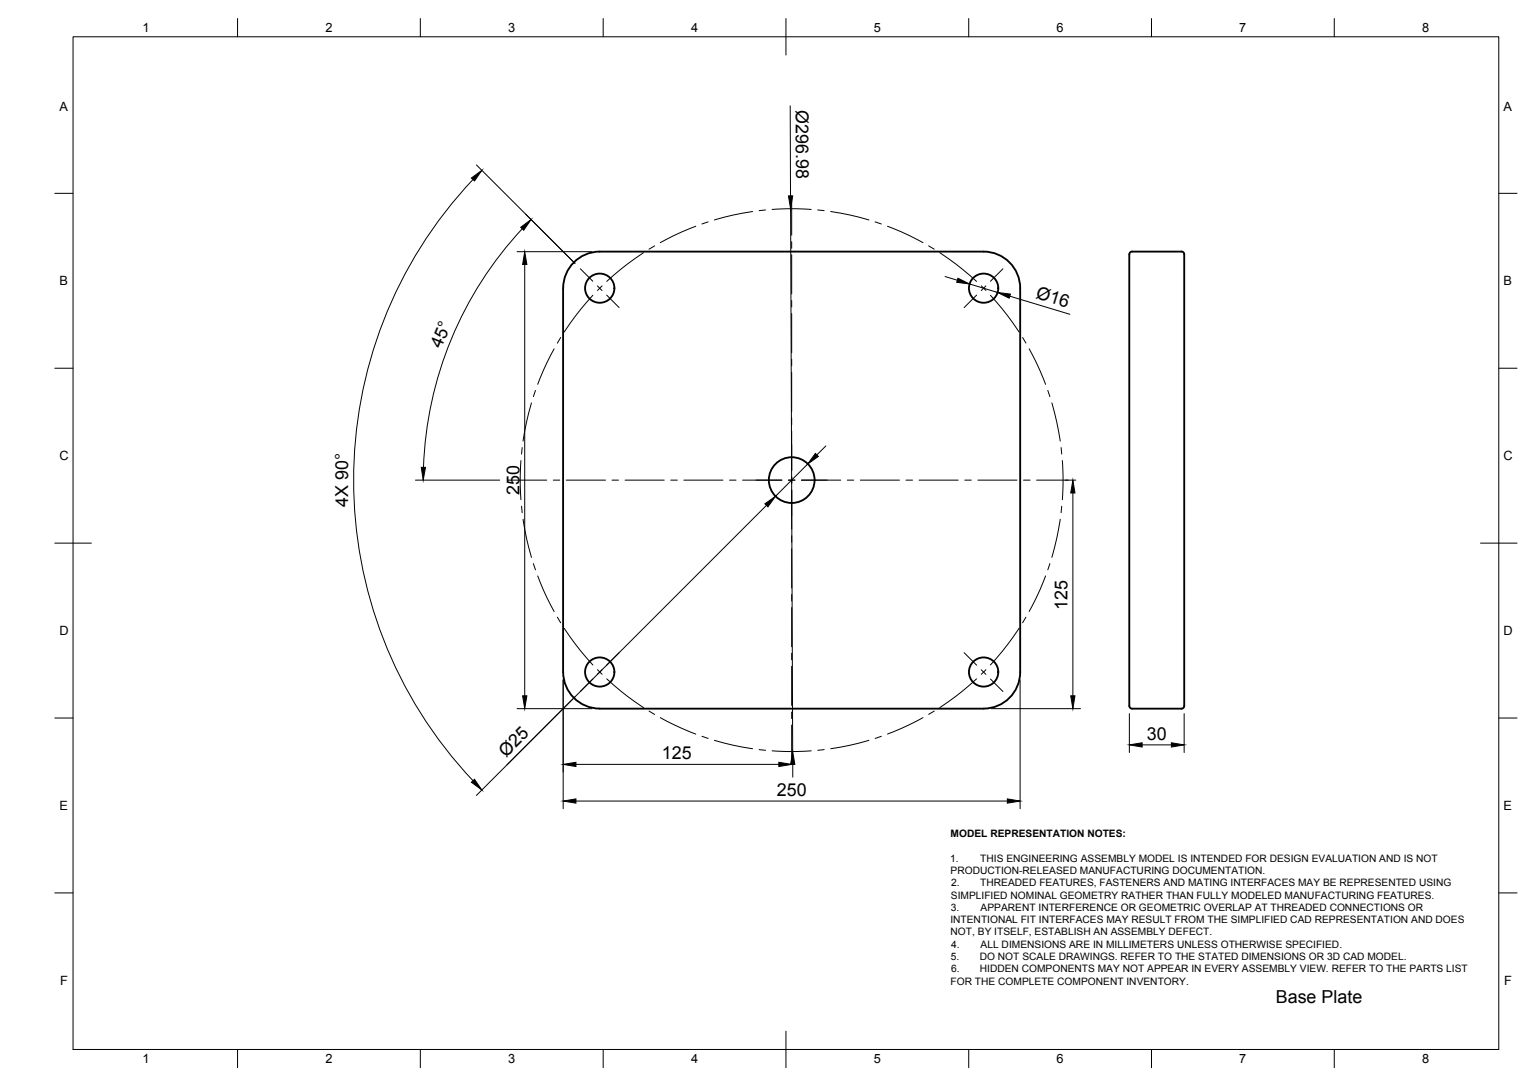
ISO-10303-21;
HEADER;
/* Generated by software containing ST-Developer
 * from STEP Tools, Inc. (www.steptools.com) 
 */

FILE_DESCRIPTION(
/* description */ ('STEP AP214'),
/* implementation_level */ '2;1');

FILE_NAME(
/* name */ 'BASE PLATE.step',
/* time_stamp */ '2026-10-06T11:20:11-07:00',
/* author */ (''),
/* organization */ (''),
/* preprocessor_version */ 'ST-DEVELOPER v20.2',
/* originating_system */ 'Autodesk Translation Framework v15.15.0.0',
/* authorisation */ '');

FILE_SCHEMA (('AUTOMOTIVE_DESIGN { 1 0 10303 214 3 1 1 }'));
ENDSEC;

DATA;
#10=MECHANICAL_DESIGN_GEOMETRIC_PRESENTATION_REPRESENTATION('',(#47),#2840);
#35=SHAPE_REPRESENTATION_RELATIONSHIP('SRR','None',#2866,#41);
#41=ADVANCED_BREP_SHAPE_REPRESENTATION('',(#53),#2834);
#47=STYLED_ITEM('',(#2905),#53);
#53=MANIFOLD_SOLID_BREP('Body1',#1547);
#59=TOROIDAL_SURFACE('',#1663,18.5,1.5);
#60=TOROIDAL_SURFACE('',#1670,18.5,1.5);
#61=TOROIDAL_SURFACE('',#1672,18.5,1.5);
#62=TOROIDAL_SURFACE('',#1678,18.5,1.5);
#63=TOROIDAL_SURFACE('',#1679,18.5,1.5);
#64=TOROIDAL_SURFACE('',#1686,18.5,1.5);
#65=TOROIDAL_SURFACE('',#1688,18.5,1.5);
#66=TOROIDAL_SURFACE('',#1694,18.5,1.5);
#70=FACE_BOUND('',#226,.T.);
#71=FACE_BOUND('',#227,.T.);
#72=FACE_BOUND('',#228,.T.);
#73=FACE_BOUND('',#229,.T.);
#74=FACE_BOUND('',#230,.T.);
#75=FACE_BOUND('',#232,.T.);
#76=FACE_BOUND('',#233,.T.);
#77=FACE_BOUND('',#234,.T.);
#78=FACE_BOUND('',#235,.T.);
#98=PLANE('',#1637);
#99=PLANE('',#1638);
#100=PLANE('',#1639);
#101=PLANE('',#1640);
#102=PLANE('',#1641);
#103=PLANE('',#1646);
#104=PLANE('',#1695);
#126=FACE_OUTER_BOUND('',#216,.T.);
#127=FACE_OUTER_BOUND('',#217,.T.);
#128=FACE_OUTER_BOUND('',#218,.T.);
#129=FACE_OUTER_BOUND('',#219,.T.);
#130=FACE_OUTER_BOUND('',#220,.T.);
#131=FACE_OUTER_BOUND('',#221,.T.);
#132=FACE_OUTER_BOUND('',#222,.T.);
#133=FACE_OUTER_BOUND('',#223,.T.);
#134=FACE_OUTER_BOUND('',#224,.T.);
#135=FACE_OUTER_BOUND('',#225,.T.);
#136=FACE_OUTER_BOUND('',#231,.T.);
#137=FACE_OUTER_BOUND('',#236,.T.);
#138=FACE_OUTER_BOUND('',#237,.T.);
#139=FACE_OUTER_BOUND('',#238,.T.);
#140=FACE_OUTER_BOUND('',#239,.T.);
#141=FACE_OUTER_BOUND('',#240,.T.);
#142=FACE_OUTER_BOUND('',#241,.T.);
#143=FACE_OUTER_BOUND('',#242,.T.);
#144=FACE_OUTER_BOUND('',#243,.T.);
#145=FACE_OUTER_BOUND('',#244,.T.);
#146=FACE_OUTER_BOUND('',#245,.T.);
#147=FACE_OUTER_BOUND('',#246,.T.);
#148=FACE_OUTER_BOUND('',#247,.T.);
#149=FACE_OUTER_BOUND('',#248,.T.);
#150=FACE_OUTER_BOUND('',#249,.T.);
#151=FACE_OUTER_BOUND('',#250,.T.);
#152=FACE_OUTER_BOUND('',#251,.T.);
#153=FACE_OUTER_BOUND('',#252,.T.);
#154=FACE_OUTER_BOUND('',#253,.T.);
#155=FACE_OUTER_BOUND('',#254,.T.);
#156=FACE_OUTER_BOUND('',#255,.T.);
#157=FACE_OUTER_BOUND('',#256,.T.);
#216=EDGE_LOOP('',(#984,#985,#986,#987));
#217=EDGE_LOOP('',(#988,#989,#990,#991));
#218=EDGE_LOOP('',(#992,#993,#994,#995));
#219=EDGE_LOOP('',(#996,#997,#998,#999));
#220=EDGE_LOOP('',(#1000,#1001,#1002,#1003));
#221=EDGE_LOOP('',(#1004,#1005,#1006,#1007));
#222=EDGE_LOOP('',(#1008,#1009,#1010,#1011));
#223=EDGE_LOOP('',(#1012,#1013,#1014,#1015));
#224=EDGE_LOOP('',(#1016,#1017,#1018,#1019));
#225=EDGE_LOOP('',(#1020,#1021,#1022,#1023,#1024,#1025,#1026,#1027));
#226=EDGE_LOOP('',(#1028));
#227=EDGE_LOOP('',(#1029));
#228=EDGE_LOOP('',(#1030));
#229=EDGE_LOOP('',(#1031));
#230=EDGE_LOOP('',(#1032));
#231=EDGE_LOOP('',(#1033,#1034,#1035,#1036,#1037,#1038,#1039,#1040));
#232=EDGE_LOOP('',(#1041));
#233=EDGE_LOOP('',(#1042));
#234=EDGE_LOOP('',(#1043));
#235=EDGE_LOOP('',(#1044));
#236=EDGE_LOOP('',(#1045,#1046,#1047,#1048));
#237=EDGE_LOOP('',(#1049,#1050,#1051,#1052));
#238=EDGE_LOOP('',(#1053,#1054,#1055,#1056));
#239=EDGE_LOOP('',(#1057,#1058,#1059,#1060));
#240=EDGE_LOOP('',(#1061,#1062,#1063,#1064));
#241=EDGE_LOOP('',(#1065,#1066,#1067,#1068));
#242=EDGE_LOOP('',(#1069,#1070,#1071,#1072));
#243=EDGE_LOOP('',(#1073,#1074,#1075,#1076));
#244=EDGE_LOOP('',(#1077,#1078,#1079,#1080));
#245=EDGE_LOOP('',(#1081,#1082,#1083,#1084));
#246=EDGE_LOOP('',(#1085,#1086,#1087,#1088));
#247=EDGE_LOOP('',(#1089,#1090,#1091,#1092));
#248=EDGE_LOOP('',(#1093,#1094,#1095,#1096));
#249=EDGE_LOOP('',(#1097,#1098,#1099,#1100));
#250=EDGE_LOOP('',(#1101,#1102,#1103,#1104));
#251=EDGE_LOOP('',(#1105,#1106,#1107,#1108));
#252=EDGE_LOOP('',(#1109,#1110,#1111,#1112));
#253=EDGE_LOOP('',(#1113,#1114,#1115,#1116));
#254=EDGE_LOOP('',(#1117,#1118,#1119,#1120));
#255=EDGE_LOOP('',(#1121,#1122,#1123,#1124));
#256=EDGE_LOOP('',(#1125));
#334=LINE('',#2382,#427);
#335=LINE('',#2388,#428);
#336=LINE('',#2394,#429);
#337=LINE('',#2400,#430);
#338=LINE('',#2406,#431);
#339=LINE('',#2411,#432);
#340=LINE('',#2413,#433);
#341=LINE('',#2415,#434);
#342=LINE('',#2416,#435);
#343=LINE('',#2420,#436);
#344=LINE('',#2422,#437);
#345=LINE('',#2424,#438);
#346=LINE('',#2425,#439);
#347=LINE('',#2429,#440);
#348=LINE('',#2431,#441);
#349=LINE('',#2433,#442);
#350=LINE('',#2434,#443);
#351=LINE('',#2438,#444);
#352=LINE('',#2440,#445);
#353=LINE('',#2442,#446);
#354=LINE('',#2443,#447);
#355=LINE('',#2447,#448);
#356=LINE('',#2451,#449);
#357=LINE('',#2455,#450);
#358=LINE('',#2459,#451);
#359=LINE('',#2464,#452);
#360=LINE('',#2468,#453);
#361=LINE('',#2472,#454);
#362=LINE('',#2476,#455);
#427=VECTOR('',#1849,12.5000000000002);
#428=VECTOR('',#1856,8.00000000000001);
#429=VECTOR('',#1863,8.00000000000001);
#430=VECTOR('',#1870,8.00000000000001);
#431=VECTOR('',#1877,8.00000000000001);
#432=VECTOR('',#1882,1000.);
#433=VECTOR('',#1883,1000.);
#434=VECTOR('',#1884,1000.);
#435=VECTOR('',#1885,1000.);
#436=VECTOR('',#1888,1000.);
#437=VECTOR('',#1889,1000.);
#438=VECTOR('',#1890,1000.);
#439=VECTOR('',#1891,1000.);
#440=VECTOR('',#1894,1000.);
#441=VECTOR('',#1895,1000.);
#442=VECTOR('',#1896,1000.);
#443=VECTOR('',#1897,1000.);
#444=VECTOR('',#1900,1000.);
#445=VECTOR('',#1901,1000.);
#446=VECTOR('',#1902,1000.);
#447=VECTOR('',#1903,1000.);
#448=VECTOR('',#1906,1000.);
#449=VECTOR('',#1909,1000.);
#450=VECTOR('',#1912,1000.);
#451=VECTOR('',#1915,1000.);
#452=VECTOR('',#1920,1000.);
#453=VECTOR('',#1923,1000.);
#454=VECTOR('',#1926,1000.);
#455=VECTOR('',#1929,1000.);
#520=CIRCLE('',#1623,12.5000000000002);
#521=CIRCLE('',#1624,12.5000000000002);
#522=CIRCLE('',#1626,8.00000000000001);
#523=CIRCLE('',#1627,8.00000000000001);
#524=CIRCLE('',#1629,8.00000000000001);
#525=CIRCLE('',#1630,8.00000000000001);
#526=CIRCLE('',#1632,8.00000000000001);
#527=CIRCLE('',#1633,8.00000000000001);
#528=CIRCLE('',#1635,8.00000000000001);
#529=CIRCLE('',#1636,8.00000000000001);
#530=CIRCLE('',#1642,18.5);
#531=CIRCLE('',#1643,18.5);
#532=CIRCLE('',#1644,18.5);
#533=CIRCLE('',#1645,18.5);
#534=CIRCLE('',#1647,18.5);
#535=CIRCLE('',#1648,18.5);
#536=CIRCLE('',#1649,18.5);
#537=CIRCLE('',#1650,18.5);
#538=CIRCLE('',#1652,20.);
#539=CIRCLE('',#1653,20.);
#540=CIRCLE('',#1655,20.);
#541=CIRCLE('',#1656,20.);
#542=CIRCLE('',#1658,20.);
#543=CIRCLE('',#1659,20.);
#544=CIRCLE('',#1661,20.);
#545=CIRCLE('',#1662,20.);
#546=CIRCLE('',#1664,1.5);
#547=CIRCLE('',#1665,1.50000000000006);
#548=CIRCLE('',#1667,1.50000000000006);
#549=CIRCLE('',#1669,1.5);
#550=CIRCLE('',#1671,1.5);
#551=CIRCLE('',#1673,1.50000000000006);
#552=CIRCLE('',#1675,1.5);
#553=CIRCLE('',#1677,1.50000000000006);
#554=CIRCLE('',#1680,1.5);
#555=CIRCLE('',#1681,1.50000000000006);
#556=CIRCLE('',#1683,1.50000000000006);
#557=CIRCLE('',#1685,1.5);
#558=CIRCLE('',#1687,1.5);
#559=CIRCLE('',#1689,1.50000000000006);
#560=CIRCLE('',#1691,1.5);
#561=CIRCLE('',#1693,1.50000000000006);
#638=VERTEX_POINT('',#2379);
#639=VERTEX_POINT('',#2381);
#640=VERTEX_POINT('',#2385);
#641=VERTEX_POINT('',#2387);
#642=VERTEX_POINT('',#2391);
#643=VERTEX_POINT('',#2393);
#644=VERTEX_POINT('',#2397);
#645=VERTEX_POINT('',#2399);
#646=VERTEX_POINT('',#2403);
#647=VERTEX_POINT('',#2405);
#648=VERTEX_POINT('',#2409);
#649=VERTEX_POINT('',#2410);
#650=VERTEX_POINT('',#2412);
#651=VERTEX_POINT('',#2414);
#652=VERTEX_POINT('',#2418);
#653=VERTEX_POINT('',#2419);
#654=VERTEX_POINT('',#2421);
#655=VERTEX_POINT('',#2423);
#656=VERTEX_POINT('',#2427);
#657=VERTEX_POINT('',#2428);
#658=VERTEX_POINT('',#2430);
#659=VERTEX_POINT('',#2432);
#660=VERTEX_POINT('',#2436);
#661=VERTEX_POINT('',#2437);
#662=VERTEX_POINT('',#2439);
#663=VERTEX_POINT('',#2441);
#664=VERTEX_POINT('',#2445);
#665=VERTEX_POINT('',#2446);
#666=VERTEX_POINT('',#2448);
#667=VERTEX_POINT('',#2450);
#668=VERTEX_POINT('',#2452);
#669=VERTEX_POINT('',#2454);
#670=VERTEX_POINT('',#2456);
#671=VERTEX_POINT('',#2458);
#672=VERTEX_POINT('',#2462);
#673=VERTEX_POINT('',#2463);
#674=VERTEX_POINT('',#2465);
#675=VERTEX_POINT('',#2467);
#676=VERTEX_POINT('',#2469);
#677=VERTEX_POINT('',#2471);
#678=VERTEX_POINT('',#2473);
#679=VERTEX_POINT('',#2475);
#773=EDGE_CURVE('',#638,#638,#520,.T.);
#774=EDGE_CURVE('',#638,#639,#334,.T.);
#775=EDGE_CURVE('',#639,#639,#521,.T.);
#776=EDGE_CURVE('',#640,#640,#522,.T.);
#777=EDGE_CURVE('',#640,#641,#335,.T.);
#778=EDGE_CURVE('',#641,#641,#523,.T.);
#779=EDGE_CURVE('',#642,#642,#524,.T.);
#780=EDGE_CURVE('',#642,#643,#336,.T.);
#781=EDGE_CURVE('',#643,#643,#525,.T.);
#782=EDGE_CURVE('',#644,#644,#526,.T.);
#783=EDGE_CURVE('',#644,#645,#337,.T.);
#784=EDGE_CURVE('',#645,#645,#527,.T.);
#785=EDGE_CURVE('',#646,#646,#528,.T.);
#786=EDGE_CURVE('',#646,#647,#338,.T.);
#787=EDGE_CURVE('',#647,#647,#529,.T.);
#788=EDGE_CURVE('',#648,#649,#339,.T.);
#789=EDGE_CURVE('',#649,#650,#340,.T.);
#790=EDGE_CURVE('',#650,#651,#341,.T.);
#791=EDGE_CURVE('',#651,#648,#342,.T.);
#792=EDGE_CURVE('',#652,#653,#343,.T.);
#793=EDGE_CURVE('',#653,#654,#344,.T.);
#794=EDGE_CURVE('',#654,#655,#345,.T.);
#795=EDGE_CURVE('',#655,#652,#346,.T.);
#796=EDGE_CURVE('',#656,#657,#347,.T.);
#797=EDGE_CURVE('',#657,#658,#348,.T.);
#798=EDGE_CURVE('',#658,#659,#349,.T.);
#799=EDGE_CURVE('',#659,#656,#350,.T.);
#800=EDGE_CURVE('',#660,#661,#351,.T.);
#801=EDGE_CURVE('',#661,#662,#352,.T.);
#802=EDGE_CURVE('',#662,#663,#353,.T.);
#803=EDGE_CURVE('',#663,#660,#354,.T.);
#804=EDGE_CURVE('',#664,#665,#355,.T.);
#805=EDGE_CURVE('',#665,#666,#530,.T.);
#806=EDGE_CURVE('',#666,#667,#356,.T.);
#807=EDGE_CURVE('',#667,#668,#531,.T.);
#808=EDGE_CURVE('',#668,#669,#357,.T.);
#809=EDGE_CURVE('',#669,#670,#532,.T.);
#810=EDGE_CURVE('',#670,#671,#358,.T.);
#811=EDGE_CURVE('',#671,#664,#533,.T.);
#812=EDGE_CURVE('',#672,#673,#359,.T.);
#813=EDGE_CURVE('',#673,#674,#534,.T.);
#814=EDGE_CURVE('',#674,#675,#360,.T.);
#815=EDGE_CURVE('',#675,#676,#535,.T.);
#816=EDGE_CURVE('',#676,#677,#361,.T.);
#817=EDGE_CURVE('',#677,#678,#536,.T.);
#818=EDGE_CURVE('',#678,#679,#362,.T.);
#819=EDGE_CURVE('',#679,#672,#537,.T.);
#820=EDGE_CURVE('',#654,#657,#538,.T.);
#821=EDGE_CURVE('',#656,#655,#539,.T.);
#822=EDGE_CURVE('',#650,#653,#540,.T.);
#823=EDGE_CURVE('',#652,#651,#541,.T.);
#824=EDGE_CURVE('',#660,#649,#542,.T.);
#825=EDGE_CURVE('',#648,#661,#543,.T.);
#826=EDGE_CURVE('',#658,#663,#544,.T.);
#827=EDGE_CURVE('',#662,#659,#545,.T.);
#828=EDGE_CURVE('',#653,#677,#546,.T.);
#829=EDGE_CURVE('',#678,#650,#547,.T.);
#830=EDGE_CURVE('',#679,#649,#548,.T.);
#831=EDGE_CURVE('',#654,#676,#549,.T.);
#832=EDGE_CURVE('',#672,#660,#550,.T.);
#833=EDGE_CURVE('',#657,#675,#551,.T.);
#834=EDGE_CURVE('',#673,#663,#552,.T.);
#835=EDGE_CURVE('',#658,#674,#553,.T.);
#836=EDGE_CURVE('',#661,#669,#554,.T.);
#837=EDGE_CURVE('',#670,#648,#555,.T.);
#838=EDGE_CURVE('',#671,#651,#556,.T.);
#839=EDGE_CURVE('',#662,#668,#557,.T.);
#840=EDGE_CURVE('',#664,#652,#558,.T.);
#841=EDGE_CURVE('',#659,#667,#559,.T.);
#842=EDGE_CURVE('',#665,#655,#560,.T.);
#843=EDGE_CURVE('',#656,#666,#561,.T.);
#984=ORIENTED_EDGE('',*,*,#773,.F.);
#985=ORIENTED_EDGE('',*,*,#774,.T.);
#986=ORIENTED_EDGE('',*,*,#775,.T.);
#987=ORIENTED_EDGE('',*,*,#774,.F.);
#988=ORIENTED_EDGE('',*,*,#776,.F.);
#989=ORIENTED_EDGE('',*,*,#777,.T.);
#990=ORIENTED_EDGE('',*,*,#778,.T.);
#991=ORIENTED_EDGE('',*,*,#777,.F.);
#992=ORIENTED_EDGE('',*,*,#779,.F.);
#993=ORIENTED_EDGE('',*,*,#780,.T.);
#994=ORIENTED_EDGE('',*,*,#781,.T.);
#995=ORIENTED_EDGE('',*,*,#780,.F.);
#996=ORIENTED_EDGE('',*,*,#782,.F.);
#997=ORIENTED_EDGE('',*,*,#783,.T.);
#998=ORIENTED_EDGE('',*,*,#784,.T.);
#999=ORIENTED_EDGE('',*,*,#783,.F.);
#1000=ORIENTED_EDGE('',*,*,#785,.F.);
#1001=ORIENTED_EDGE('',*,*,#786,.T.);
#1002=ORIENTED_EDGE('',*,*,#787,.T.);
#1003=ORIENTED_EDGE('',*,*,#786,.F.);
#1004=ORIENTED_EDGE('',*,*,#788,.T.);
#1005=ORIENTED_EDGE('',*,*,#789,.T.);
#1006=ORIENTED_EDGE('',*,*,#790,.T.);
#1007=ORIENTED_EDGE('',*,*,#791,.T.);
#1008=ORIENTED_EDGE('',*,*,#792,.T.);
#1009=ORIENTED_EDGE('',*,*,#793,.T.);
#1010=ORIENTED_EDGE('',*,*,#794,.T.);
#1011=ORIENTED_EDGE('',*,*,#795,.T.);
#1012=ORIENTED_EDGE('',*,*,#796,.T.);
#1013=ORIENTED_EDGE('',*,*,#797,.T.);
#1014=ORIENTED_EDGE('',*,*,#798,.T.);
#1015=ORIENTED_EDGE('',*,*,#799,.T.);
#1016=ORIENTED_EDGE('',*,*,#800,.T.);
#1017=ORIENTED_EDGE('',*,*,#801,.T.);
#1018=ORIENTED_EDGE('',*,*,#802,.T.);
#1019=ORIENTED_EDGE('',*,*,#803,.T.);
#1020=ORIENTED_EDGE('',*,*,#804,.T.);
#1021=ORIENTED_EDGE('',*,*,#805,.T.);
#1022=ORIENTED_EDGE('',*,*,#806,.T.);
#1023=ORIENTED_EDGE('',*,*,#807,.T.);
#1024=ORIENTED_EDGE('',*,*,#808,.T.);
#1025=ORIENTED_EDGE('',*,*,#809,.T.);
#1026=ORIENTED_EDGE('',*,*,#810,.T.);
#1027=ORIENTED_EDGE('',*,*,#811,.T.);
#1028=ORIENTED_EDGE('',*,*,#778,.F.);
#1029=ORIENTED_EDGE('',*,*,#781,.F.);
#1030=ORIENTED_EDGE('',*,*,#784,.F.);
#1031=ORIENTED_EDGE('',*,*,#787,.F.);
#1032=ORIENTED_EDGE('',*,*,#775,.F.);
#1033=ORIENTED_EDGE('',*,*,#812,.T.);
#1034=ORIENTED_EDGE('',*,*,#813,.T.);
#1035=ORIENTED_EDGE('',*,*,#814,.T.);
#1036=ORIENTED_EDGE('',*,*,#815,.T.);
#1037=ORIENTED_EDGE('',*,*,#816,.T.);
#1038=ORIENTED_EDGE('',*,*,#817,.T.);
#1039=ORIENTED_EDGE('',*,*,#818,.T.);
#1040=ORIENTED_EDGE('',*,*,#819,.T.);
#1041=ORIENTED_EDGE('',*,*,#776,.T.);
#1042=ORIENTED_EDGE('',*,*,#779,.T.);
#1043=ORIENTED_EDGE('',*,*,#782,.T.);
#1044=ORIENTED_EDGE('',*,*,#785,.T.);
#1045=ORIENTED_EDGE('',*,*,#794,.F.);
#1046=ORIENTED_EDGE('',*,*,#820,.T.);
#1047=ORIENTED_EDGE('',*,*,#796,.F.);
#1048=ORIENTED_EDGE('',*,*,#821,.T.);
#1049=ORIENTED_EDGE('',*,*,#790,.F.);
#1050=ORIENTED_EDGE('',*,*,#822,.T.);
#1051=ORIENTED_EDGE('',*,*,#792,.F.);
#1052=ORIENTED_EDGE('',*,*,#823,.T.);
#1053=ORIENTED_EDGE('',*,*,#800,.F.);
#1054=ORIENTED_EDGE('',*,*,#824,.T.);
#1055=ORIENTED_EDGE('',*,*,#788,.F.);
#1056=ORIENTED_EDGE('',*,*,#825,.T.);
#1057=ORIENTED_EDGE('',*,*,#798,.F.);
#1058=ORIENTED_EDGE('',*,*,#826,.T.);
#1059=ORIENTED_EDGE('',*,*,#802,.F.);
#1060=ORIENTED_EDGE('',*,*,#827,.T.);
#1061=ORIENTED_EDGE('',*,*,#828,.F.);
#1062=ORIENTED_EDGE('',*,*,#822,.F.);
#1063=ORIENTED_EDGE('',*,*,#829,.F.);
#1064=ORIENTED_EDGE('',*,*,#817,.F.);
#1065=ORIENTED_EDGE('',*,*,#829,.T.);
#1066=ORIENTED_EDGE('',*,*,#789,.F.);
#1067=ORIENTED_EDGE('',*,*,#830,.F.);
#1068=ORIENTED_EDGE('',*,*,#818,.F.);
#1069=ORIENTED_EDGE('',*,*,#828,.T.);
#1070=ORIENTED_EDGE('',*,*,#816,.F.);
#1071=ORIENTED_EDGE('',*,*,#831,.F.);
#1072=ORIENTED_EDGE('',*,*,#793,.F.);
#1073=ORIENTED_EDGE('',*,*,#830,.T.);
#1074=ORIENTED_EDGE('',*,*,#824,.F.);
#1075=ORIENTED_EDGE('',*,*,#832,.F.);
#1076=ORIENTED_EDGE('',*,*,#819,.F.);
#1077=ORIENTED_EDGE('',*,*,#831,.T.);
#1078=ORIENTED_EDGE('',*,*,#815,.F.);
#1079=ORIENTED_EDGE('',*,*,#833,.F.);
#1080=ORIENTED_EDGE('',*,*,#820,.F.);
#1081=ORIENTED_EDGE('',*,*,#832,.T.);
#1082=ORIENTED_EDGE('',*,*,#803,.F.);
#1083=ORIENTED_EDGE('',*,*,#834,.F.);
#1084=ORIENTED_EDGE('',*,*,#812,.F.);
#1085=ORIENTED_EDGE('',*,*,#833,.T.);
#1086=ORIENTED_EDGE('',*,*,#814,.F.);
#1087=ORIENTED_EDGE('',*,*,#835,.F.);
#1088=ORIENTED_EDGE('',*,*,#797,.F.);
#1089=ORIENTED_EDGE('',*,*,#834,.T.);
#1090=ORIENTED_EDGE('',*,*,#826,.F.);
#1091=ORIENTED_EDGE('',*,*,#835,.T.);
#1092=ORIENTED_EDGE('',*,*,#813,.F.);
#1093=ORIENTED_EDGE('',*,*,#836,.F.);
#1094=ORIENTED_EDGE('',*,*,#825,.F.);
#1095=ORIENTED_EDGE('',*,*,#837,.F.);
#1096=ORIENTED_EDGE('',*,*,#809,.F.);
#1097=ORIENTED_EDGE('',*,*,#837,.T.);
#1098=ORIENTED_EDGE('',*,*,#791,.F.);
#1099=ORIENTED_EDGE('',*,*,#838,.F.);
#1100=ORIENTED_EDGE('',*,*,#810,.F.);
#1101=ORIENTED_EDGE('',*,*,#836,.T.);
#1102=ORIENTED_EDGE('',*,*,#808,.F.);
#1103=ORIENTED_EDGE('',*,*,#839,.F.);
#1104=ORIENTED_EDGE('',*,*,#801,.F.);
#1105=ORIENTED_EDGE('',*,*,#838,.T.);
#1106=ORIENTED_EDGE('',*,*,#823,.F.);
#1107=ORIENTED_EDGE('',*,*,#840,.F.);
#1108=ORIENTED_EDGE('',*,*,#811,.F.);
#1109=ORIENTED_EDGE('',*,*,#839,.T.);
#1110=ORIENTED_EDGE('',*,*,#807,.F.);
#1111=ORIENTED_EDGE('',*,*,#841,.F.);
#1112=ORIENTED_EDGE('',*,*,#827,.F.);
#1113=ORIENTED_EDGE('',*,*,#840,.T.);
#1114=ORIENTED_EDGE('',*,*,#795,.F.);
#1115=ORIENTED_EDGE('',*,*,#842,.F.);
#1116=ORIENTED_EDGE('',*,*,#804,.F.);
#1117=ORIENTED_EDGE('',*,*,#841,.T.);
#1118=ORIENTED_EDGE('',*,*,#806,.F.);
#1119=ORIENTED_EDGE('',*,*,#843,.F.);
#1120=ORIENTED_EDGE('',*,*,#799,.F.);
#1121=ORIENTED_EDGE('',*,*,#842,.T.);
#1122=ORIENTED_EDGE('',*,*,#821,.F.);
#1123=ORIENTED_EDGE('',*,*,#843,.T.);
#1124=ORIENTED_EDGE('',*,*,#805,.F.);
#1125=ORIENTED_EDGE('',*,*,#773,.T.);
#1406=CYLINDRICAL_SURFACE('',#1622,12.5000000000002);
#1407=CYLINDRICAL_SURFACE('',#1625,8.00000000000001);
#1408=CYLINDRICAL_SURFACE('',#1628,8.00000000000001);
#1409=CYLINDRICAL_SURFACE('',#1631,8.00000000000001);
#1410=CYLINDRICAL_SURFACE('',#1634,8.00000000000001);
#1411=CYLINDRICAL_SURFACE('',#1651,20.);
#1412=CYLINDRICAL_SURFACE('',#1654,20.);
#1413=CYLINDRICAL_SURFACE('',#1657,20.);
#1414=CYLINDRICAL_SURFACE('',#1660,20.);
#1415=CYLINDRICAL_SURFACE('',#1666,1.50000000000006);
#1416=CYLINDRICAL_SURFACE('',#1668,1.5);
#1417=CYLINDRICAL_SURFACE('',#1674,1.5);
#1418=CYLINDRICAL_SURFACE('',#1676,1.50000000000006);
#1419=CYLINDRICAL_SURFACE('',#1682,1.50000000000006);
#1420=CYLINDRICAL_SURFACE('',#1684,1.5);
#1421=CYLINDRICAL_SURFACE('',#1690,1.5);
#1422=CYLINDRICAL_SURFACE('',#1692,1.50000000000006);
#1457=ADVANCED_FACE('',(#126),#1406,.F.);
#1458=ADVANCED_FACE('',(#127),#1407,.F.);
#1459=ADVANCED_FACE('',(#128),#1408,.F.);
#1460=ADVANCED_FACE('',(#129),#1409,.F.);
#1461=ADVANCED_FACE('',(#130),#1410,.F.);
#1462=ADVANCED_FACE('',(#131),#98,.T.);
#1463=ADVANCED_FACE('',(#132),#99,.T.);
#1464=ADVANCED_FACE('',(#133),#100,.F.);
#1465=ADVANCED_FACE('',(#134),#101,.F.);
#1466=ADVANCED_FACE('',(#135,#70,#71,#72,#73,#74),#102,.T.);
#1467=ADVANCED_FACE('',(#136,#75,#76,#77,#78),#103,.F.);
#1468=ADVANCED_FACE('',(#137),#1411,.T.);
#1469=ADVANCED_FACE('',(#138),#1412,.T.);
#1470=ADVANCED_FACE('',(#139),#1413,.T.);
#1471=ADVANCED_FACE('',(#140),#1414,.T.);
#1472=ADVANCED_FACE('',(#141),#59,.T.);
#1473=ADVANCED_FACE('',(#142),#1415,.T.);
#1474=ADVANCED_FACE('',(#143),#1416,.T.);
#1475=ADVANCED_FACE('',(#144),#60,.T.);
#1476=ADVANCED_FACE('',(#145),#61,.T.);
#1477=ADVANCED_FACE('',(#146),#1417,.T.);
#1478=ADVANCED_FACE('',(#147),#1418,.T.);
#1479=ADVANCED_FACE('',(#148),#62,.T.);
#1480=ADVANCED_FACE('',(#149),#63,.T.);
#1481=ADVANCED_FACE('',(#150),#1419,.T.);
#1482=ADVANCED_FACE('',(#151),#1420,.T.);
#1483=ADVANCED_FACE('',(#152),#64,.T.);
#1484=ADVANCED_FACE('',(#153),#65,.T.);
#1485=ADVANCED_FACE('',(#154),#1421,.T.);
#1486=ADVANCED_FACE('',(#155),#1422,.T.);
#1487=ADVANCED_FACE('',(#156),#66,.T.);
#1488=ADVANCED_FACE('',(#157),#104,.T.);
#1547=CLOSED_SHELL('',(#1457,#1458,#1459,#1460,#1461,#1462,#1463,#1464,
#1465,#1466,#1467,#1468,#1469,#1470,#1471,#1472,#1473,#1474,#1475,#1476,
#1477,#1478,#1479,#1480,#1481,#1482,#1483,#1484,#1485,#1486,#1487,#1488));
#1621=AXIS2_PLACEMENT_3D('',#2377,#1843,#1844);
#1622=AXIS2_PLACEMENT_3D('',#2378,#1845,#1846);
#1623=AXIS2_PLACEMENT_3D('',#2380,#1847,#1848);
#1624=AXIS2_PLACEMENT_3D('',#2383,#1850,#1851);
#1625=AXIS2_PLACEMENT_3D('',#2384,#1852,#1853);
#1626=AXIS2_PLACEMENT_3D('',#2386,#1854,#1855);
#1627=AXIS2_PLACEMENT_3D('',#2389,#1857,#1858);
#1628=AXIS2_PLACEMENT_3D('',#2390,#1859,#1860);
#1629=AXIS2_PLACEMENT_3D('',#2392,#1861,#1862);
#1630=AXIS2_PLACEMENT_3D('',#2395,#1864,#1865);
#1631=AXIS2_PLACEMENT_3D('',#2396,#1866,#1867);
#1632=AXIS2_PLACEMENT_3D('',#2398,#1868,#1869);
#1633=AXIS2_PLACEMENT_3D('',#2401,#1871,#1872);
#1634=AXIS2_PLACEMENT_3D('',#2402,#1873,#1874);
#1635=AXIS2_PLACEMENT_3D('',#2404,#1875,#1876);
#1636=AXIS2_PLACEMENT_3D('',#2407,#1878,#1879);
#1637=AXIS2_PLACEMENT_3D('',#2408,#1880,#1881);
#1638=AXIS2_PLACEMENT_3D('',#2417,#1886,#1887);
#1639=AXIS2_PLACEMENT_3D('',#2426,#1892,#1893);
#1640=AXIS2_PLACEMENT_3D('',#2435,#1898,#1899);
#1641=AXIS2_PLACEMENT_3D('',#2444,#1904,#1905);
#1642=AXIS2_PLACEMENT_3D('',#2449,#1907,#1908);
#1643=AXIS2_PLACEMENT_3D('',#2453,#1910,#1911);
#1644=AXIS2_PLACEMENT_3D('',#2457,#1913,#1914);
#1645=AXIS2_PLACEMENT_3D('',#2460,#1916,#1917);
#1646=AXIS2_PLACEMENT_3D('',#2461,#1918,#1919);
#1647=AXIS2_PLACEMENT_3D('',#2466,#1921,#1922);
#1648=AXIS2_PLACEMENT_3D('',#2470,#1924,#1925);
#1649=AXIS2_PLACEMENT_3D('',#2474,#1927,#1928);
#1650=AXIS2_PLACEMENT_3D('',#2477,#1930,#1931);
#1651=AXIS2_PLACEMENT_3D('',#2478,#1932,#1933);
#1652=AXIS2_PLACEMENT_3D('',#2479,#1934,#1935);
#1653=AXIS2_PLACEMENT_3D('',#2480,#1936,#1937);
#1654=AXIS2_PLACEMENT_3D('',#2481,#1938,#1939);
#1655=AXIS2_PLACEMENT_3D('',#2482,#1940,#1941);
#1656=AXIS2_PLACEMENT_3D('',#2483,#1942,#1943);
#1657=AXIS2_PLACEMENT_3D('',#2484,#1944,#1945);
#1658=AXIS2_PLACEMENT_3D('',#2485,#1946,#1947);
#1659=AXIS2_PLACEMENT_3D('',#2486,#1948,#1949);
#1660=AXIS2_PLACEMENT_3D('',#2487,#1950,#1951);
#1661=AXIS2_PLACEMENT_3D('',#2488,#1952,#1953);
#1662=AXIS2_PLACEMENT_3D('',#2489,#1954,#1955);
#1663=AXIS2_PLACEMENT_3D('',#2490,#1956,#1957);
#1664=AXIS2_PLACEMENT_3D('',#2491,#1958,#1959);
#1665=AXIS2_PLACEMENT_3D('',#2492,#1960,#1961);
#1666=AXIS2_PLACEMENT_3D('',#2493,#1962,#1963);
#1667=AXIS2_PLACEMENT_3D('',#2494,#1964,#1965);
#1668=AXIS2_PLACEMENT_3D('',#2495,#1966,#1967);
#1669=AXIS2_PLACEMENT_3D('',#2496,#1968,#1969);
#1670=AXIS2_PLACEMENT_3D('',#2497,#1970,#1971);
#1671=AXIS2_PLACEMENT_3D('',#2498,#1972,#1973);
#1672=AXIS2_PLACEMENT_3D('',#2499,#1974,#1975);
#1673=AXIS2_PLACEMENT_3D('',#2500,#1976,#1977);
#1674=AXIS2_PLACEMENT_3D('',#2501,#1978,#1979);
#1675=AXIS2_PLACEMENT_3D('',#2502,#1980,#1981);
#1676=AXIS2_PLACEMENT_3D('',#2503,#1982,#1983);
#1677=AXIS2_PLACEMENT_3D('',#2504,#1984,#1985);
#1678=AXIS2_PLACEMENT_3D('',#2505,#1986,#1987);
#1679=AXIS2_PLACEMENT_3D('',#2506,#1988,#1989);
#1680=AXIS2_PLACEMENT_3D('',#2507,#1990,#1991);
#1681=AXIS2_PLACEMENT_3D('',#2508,#1992,#1993);
#1682=AXIS2_PLACEMENT_3D('',#2509,#1994,#1995);
#1683=AXIS2_PLACEMENT_3D('',#2510,#1996,#1997);
#1684=AXIS2_PLACEMENT_3D('',#2511,#1998,#1999);
#1685=AXIS2_PLACEMENT_3D('',#2512,#2000,#2001);
#1686=AXIS2_PLACEMENT_3D('',#2513,#2002,#2003);
#1687=AXIS2_PLACEMENT_3D('',#2514,#2004,#2005);
#1688=AXIS2_PLACEMENT_3D('',#2515,#2006,#2007);
#1689=AXIS2_PLACEMENT_3D('',#2516,#2008,#2009);
#1690=AXIS2_PLACEMENT_3D('',#2517,#2010,#2011);
#1691=AXIS2_PLACEMENT_3D('',#2518,#2012,#2013);
#1692=AXIS2_PLACEMENT_3D('',#2519,#2014,#2015);
#1693=AXIS2_PLACEMENT_3D('',#2520,#2016,#2017);
#1694=AXIS2_PLACEMENT_3D('',#2521,#2018,#2019);
#1695=AXIS2_PLACEMENT_3D('',#2522,#2020,#2021);
#1843=DIRECTION('axis',(0.,0.,1.));
#1844=DIRECTION('refdir',(1.,0.,0.));
#1845=DIRECTION('center_axis',(0.,1.,0.));
#1846=DIRECTION('ref_axis',(0.,0.,1.));
#1847=DIRECTION('center_axis',(0.,1.,0.));
#1848=DIRECTION('ref_axis',(0.,0.,1.));
#1849=DIRECTION('',(0.,1.,0.));
#1850=DIRECTION('center_axis',(0.,1.,0.));
#1851=DIRECTION('ref_axis',(0.,0.,1.));
#1852=DIRECTION('center_axis',(0.,1.,0.));
#1853=DIRECTION('ref_axis',(0.,0.,1.));
#1854=DIRECTION('center_axis',(0.,1.,0.));
#1855=DIRECTION('ref_axis',(0.,0.,1.));
#1856=DIRECTION('',(0.,1.,0.));
#1857=DIRECTION('center_axis',(0.,1.,0.));
#1858=DIRECTION('ref_axis',(0.,0.,1.));
#1859=DIRECTION('center_axis',(0.,1.,0.));
#1860=DIRECTION('ref_axis',(0.,0.,1.));
#1861=DIRECTION('center_axis',(0.,1.,0.));
#1862=DIRECTION('ref_axis',(0.,0.,1.));
#1863=DIRECTION('',(0.,1.,0.));
#1864=DIRECTION('center_axis',(0.,1.,0.));
#1865=DIRECTION('ref_axis',(0.,0.,1.));
#1866=DIRECTION('center_axis',(0.,1.,0.));
#1867=DIRECTION('ref_axis',(0.,0.,1.));
#1868=DIRECTION('center_axis',(0.,1.,0.));
#1869=DIRECTION('ref_axis',(0.,0.,1.));
#1870=DIRECTION('',(0.,1.,0.));
#1871=DIRECTION('center_axis',(0.,1.,0.));
#1872=DIRECTION('ref_axis',(0.,0.,1.));
#1873=DIRECTION('center_axis',(0.,1.,0.));
#1874=DIRECTION('ref_axis',(0.,0.,1.));
#1875=DIRECTION('center_axis',(0.,1.,0.));
#1876=DIRECTION('ref_axis',(0.,0.,1.));
#1877=DIRECTION('',(0.,1.,0.));
#1878=DIRECTION('center_axis',(0.,1.,0.));
#1879=DIRECTION('ref_axis',(0.,0.,1.));
#1880=DIRECTION('center_axis',(0.,0.,-1.));
#1881=DIRECTION('ref_axis',(-1.,0.,0.));
#1882=DIRECTION('',(0.,-1.,0.));
#1883=DIRECTION('',(-1.,0.,0.));
#1884=DIRECTION('',(0.,1.,0.));
#1885=DIRECTION('',(1.,0.,0.));
#1886=DIRECTION('center_axis',(-1.,0.,0.));
#1887=DIRECTION('ref_axis',(0.,0.,1.));
#1888=DIRECTION('',(0.,-1.,0.));
#1889=DIRECTION('',(0.,0.,1.));
#1890=DIRECTION('',(0.,1.,0.));
#1891=DIRECTION('',(0.,0.,-1.));
#1892=DIRECTION('center_axis',(0.,0.,-1.));
#1893=DIRECTION('ref_axis',(-1.,0.,0.));
#1894=DIRECTION('',(0.,-1.,0.));
#1895=DIRECTION('',(1.,0.,0.));
#1896=DIRECTION('',(0.,1.,0.));
#1897=DIRECTION('',(-1.,0.,0.));
#1898=DIRECTION('center_axis',(-1.,0.,0.));
#1899=DIRECTION('ref_axis',(0.,0.,1.));
#1900=DIRECTION('',(0.,1.,0.));
#1901=DIRECTION('',(0.,0.,1.));
#1902=DIRECTION('',(0.,-1.,0.));
#1903=DIRECTION('',(0.,0.,-1.));
#1904=DIRECTION('center_axis',(0.,1.,0.));
#1905=DIRECTION('ref_axis',(0.,0.,1.));
#1906=DIRECTION('',(0.,0.,1.));
#1907=DIRECTION('center_axis',(0.,1.,0.));
#1908=DIRECTION('ref_axis',(0.,0.,1.));
#1909=DIRECTION('',(1.,0.,0.));
#1910=DIRECTION('center_axis',(0.,1.,0.));
#1911=DIRECTION('ref_axis',(0.,0.,1.));
#1912=DIRECTION('',(0.,0.,-1.));
#1913=DIRECTION('center_axis',(0.,1.,0.));
#1914=DIRECTION('ref_axis',(0.,0.,1.));
#1915=DIRECTION('',(-1.,0.,0.));
#1916=DIRECTION('center_axis',(0.,1.,0.));
#1917=DIRECTION('ref_axis',(0.,0.,1.));
#1918=DIRECTION('center_axis',(0.,1.,0.));
#1919=DIRECTION('ref_axis',(0.,0.,1.));
#1920=DIRECTION('',(0.,0.,1.));
#1921=DIRECTION('center_axis',(0.,-1.,0.));
#1922=DIRECTION('ref_axis',(0.,0.,1.));
#1923=DIRECTION('',(-1.,0.,0.));
#1924=DIRECTION('center_axis',(0.,-1.,0.));
#1925=DIRECTION('ref_axis',(0.,0.,1.));
#1926=DIRECTION('',(0.,0.,-1.));
#1927=DIRECTION('center_axis',(0.,-1.,0.));
#1928=DIRECTION('ref_axis',(0.,0.,1.));
#1929=DIRECTION('',(1.,0.,0.));
#1930=DIRECTION('center_axis',(0.,-1.,0.));
#1931=DIRECTION('ref_axis',(0.,0.,1.));
#1932=DIRECTION('center_axis',(0.,1.,0.));
#1933=DIRECTION('ref_axis',(0.,0.,1.));
#1934=DIRECTION('center_axis',(0.,1.,0.));
#1935=DIRECTION('ref_axis',(0.,0.,1.));
#1936=DIRECTION('center_axis',(0.,-1.,0.));
#1937=DIRECTION('ref_axis',(0.,0.,1.));
#1938=DIRECTION('center_axis',(0.,-1.,0.));
#1939=DIRECTION('ref_axis',(0.,0.,-1.));
#1940=DIRECTION('center_axis',(0.,1.,0.));
#1941=DIRECTION('ref_axis',(0.,0.,1.));
#1942=DIRECTION('center_axis',(0.,-1.,0.));
#1943=DIRECTION('ref_axis',(0.,0.,1.));
#1944=DIRECTION('center_axis',(0.,1.,0.));
#1945=DIRECTION('ref_axis',(0.,0.,1.));
#1946=DIRECTION('center_axis',(0.,1.,0.));
#1947=DIRECTION('ref_axis',(0.,0.,1.));
#1948=DIRECTION('center_axis',(0.,-1.,0.));
#1949=DIRECTION('ref_axis',(0.,0.,1.));
#1950=DIRECTION('center_axis',(0.,-1.,0.));
#1951=DIRECTION('ref_axis',(0.,0.,-1.));
#1952=DIRECTION('center_axis',(0.,1.,0.));
#1953=DIRECTION('ref_axis',(0.,0.,1.));
#1954=DIRECTION('center_axis',(0.,-1.,0.));
#1955=DIRECTION('ref_axis',(0.,0.,1.));
#1956=DIRECTION('center_axis',(0.,1.,0.));
#1957=DIRECTION('ref_axis',(0.,0.,1.));
#1958=DIRECTION('center_axis',(0.,0.,1.));
#1959=DIRECTION('ref_axis',(1.,0.,0.));
#1960=DIRECTION('center_axis',(1.,0.,0.));
#1961=DIRECTION('ref_axis',(0.,0.,-1.));
#1962=DIRECTION('center_axis',(-1.,0.,0.));
#1963=DIRECTION('ref_axis',(0.,0.,1.));
#1964=DIRECTION('center_axis',(1.,0.,0.));
#1965=DIRECTION('ref_axis',(0.,0.,-1.));
#1966=DIRECTION('center_axis',(0.,0.,1.));
#1967=DIRECTION('ref_axis',(1.,0.,0.));
#1968=DIRECTION('center_axis',(0.,0.,1.));
#1969=DIRECTION('ref_axis',(1.,0.,0.));
#1970=DIRECTION('center_axis',(0.,1.,0.));
#1971=DIRECTION('ref_axis',(0.,0.,1.));
#1972=DIRECTION('center_axis',(0.,0.,1.));
#1973=DIRECTION('ref_axis',(1.,0.,0.));
#1974=DIRECTION('center_axis',(0.,1.,0.));
#1975=DIRECTION('ref_axis',(0.,0.,1.));
#1976=DIRECTION('center_axis',(1.,0.,0.));
#1977=DIRECTION('ref_axis',(0.,0.,-1.));
#1978=DIRECTION('center_axis',(0.,0.,-1.));
#1979=DIRECTION('ref_axis',(-1.,0.,0.));
#1980=DIRECTION('center_axis',(0.,0.,1.));
#1981=DIRECTION('ref_axis',(1.,0.,0.));
#1982=DIRECTION('center_axis',(1.,0.,0.));
#1983=DIRECTION('ref_axis',(0.,0.,-1.));
#1984=DIRECTION('center_axis',(1.,0.,0.));
#1985=DIRECTION('ref_axis',(0.,0.,-1.));
#1986=DIRECTION('center_axis',(0.,1.,0.));
#1987=DIRECTION('ref_axis',(0.,0.,1.));
#1988=DIRECTION('center_axis',(0.,1.,0.));
#1989=DIRECTION('ref_axis',(0.,0.,1.));
#1990=DIRECTION('center_axis',(0.,0.,1.));
#1991=DIRECTION('ref_axis',(1.,0.,0.));
#1992=DIRECTION('center_axis',(-1.,0.,0.));
#1993=DIRECTION('ref_axis',(0.,0.,1.));
#1994=DIRECTION('center_axis',(1.,0.,0.));
#1995=DIRECTION('ref_axis',(0.,0.,-1.));
#1996=DIRECTION('center_axis',(-1.,0.,0.));
#1997=DIRECTION('ref_axis',(0.,0.,1.));
#1998=DIRECTION('center_axis',(0.,0.,1.));
#1999=DIRECTION('ref_axis',(1.,0.,0.));
#2000=DIRECTION('center_axis',(0.,0.,1.));
#2001=DIRECTION('ref_axis',(1.,0.,0.));
#2002=DIRECTION('center_axis',(0.,1.,0.));
#2003=DIRECTION('ref_axis',(0.,0.,1.));
#2004=DIRECTION('center_axis',(0.,0.,1.));
#2005=DIRECTION('ref_axis',(1.,0.,0.));
#2006=DIRECTION('center_axis',(0.,1.,0.));
#2007=DIRECTION('ref_axis',(0.,0.,1.));
#2008=DIRECTION('center_axis',(-1.,0.,0.));
#2009=DIRECTION('ref_axis',(0.,0.,1.));
#2010=DIRECTION('center_axis',(0.,0.,-1.));
#2011=DIRECTION('ref_axis',(-1.,0.,0.));
#2012=DIRECTION('center_axis',(0.,0.,1.));
#2013=DIRECTION('ref_axis',(1.,0.,0.));
#2014=DIRECTION('center_axis',(-1.,0.,0.));
#2015=DIRECTION('ref_axis',(0.,0.,1.));
#2016=DIRECTION('center_axis',(-1.,0.,0.));
#2017=DIRECTION('ref_axis',(0.,0.,1.));
#2018=DIRECTION('center_axis',(0.,1.,0.));
#2019=DIRECTION('ref_axis',(0.,0.,1.));
#2020=DIRECTION('center_axis',(0.,1.,0.));
#2021=DIRECTION('ref_axis',(0.,0.,1.));
#2377=CARTESIAN_POINT('',(0.,0.,0.));
#2378=CARTESIAN_POINT('Origin',(88.4184469844746,20.,-2074.54745691296));
#2379=CARTESIAN_POINT('',(88.4184469844746,20.,-2087.04745691296));
#2380=CARTESIAN_POINT('Origin',(88.4184469844746,20.,-2074.54745691296));
#2381=CARTESIAN_POINT('',(88.4184469844746,30.,-2087.04745691296));
#2382=CARTESIAN_POINT('',(88.4184469844746,20.,-2087.04745691296));
#2383=CARTESIAN_POINT('Origin',(88.4184469844746,30.,-2074.54745691296));
#2384=CARTESIAN_POINT('Origin',(-16.5815530155254,30.,-1969.54745691296));
#2385=CARTESIAN_POINT('',(-16.5815530155254,0.,-1977.54745691296));
#2386=CARTESIAN_POINT('Origin',(-16.5815530155254,0.,-1969.54745691296));
#2387=CARTESIAN_POINT('',(-16.5815530155254,30.,-1977.54745691296));
#2388=CARTESIAN_POINT('',(-16.5815530155254,30.,-1977.54745691296));
#2389=CARTESIAN_POINT('Origin',(-16.5815530155254,30.,-1969.54745691296));
#2390=CARTESIAN_POINT('Origin',(-16.5815530155254,30.,-2179.54745691296));
#2391=CARTESIAN_POINT('',(-16.5815530155254,0.,-2187.54745691296));
#2392=CARTESIAN_POINT('Origin',(-16.5815530155254,0.,-2179.54745691296));
#2393=CARTESIAN_POINT('',(-16.5815530155254,30.,-2187.54745691296));
#2394=CARTESIAN_POINT('',(-16.5815530155254,30.,-2187.54745691296));
#2395=CARTESIAN_POINT('Origin',(-16.5815530155254,30.,-2179.54745691296));
#2396=CARTESIAN_POINT('Origin',(193.418446984475,30.,-2179.54745691296));
#2397=CARTESIAN_POINT('',(193.418446984475,0.,-2187.54745691296));
#2398=CARTESIAN_POINT('Origin',(193.418446984475,0.,-2179.54745691296));
#2399=CARTESIAN_POINT('',(193.418446984475,30.,-2187.54745691296));
#2400=CARTESIAN_POINT('',(193.418446984475,30.,-2187.54745691296));
#2401=CARTESIAN_POINT('Origin',(193.418446984475,30.,-2179.54745691296));
#2402=CARTESIAN_POINT('Origin',(193.418446984475,30.,-1969.54745691296));
#2403=CARTESIAN_POINT('',(193.418446984475,0.,-1977.54745691296));
#2404=CARTESIAN_POINT('Origin',(193.418446984475,0.,-1969.54745691296));
#2405=CARTESIAN_POINT('',(193.418446984475,30.,-1977.54745691296));
#2406=CARTESIAN_POINT('',(193.418446984475,30.,-1977.54745691296));
#2407=CARTESIAN_POINT('Origin',(193.418446984475,30.,-1969.54745691296));
#2408=CARTESIAN_POINT('Origin',(-36.5815530155254,30.,-2199.54745691296));
#2409=CARTESIAN_POINT('',(193.418446984475,28.5,-2199.54745691296));
#2410=CARTESIAN_POINT('',(193.418446984475,1.5,-2199.54745691296));
#2411=CARTESIAN_POINT('',(193.418446984475,0.,-2199.54745691296));
#2412=CARTESIAN_POINT('',(-16.5815530155254,1.5,-2199.54745691296));
#2413=CARTESIAN_POINT('',(-16.5815530155254,1.5,-2199.54745691296));
#2414=CARTESIAN_POINT('',(-16.5815530155254,28.5,-2199.54745691296));
#2415=CARTESIAN_POINT('',(-16.5815530155254,30.,-2199.54745691296));
#2416=CARTESIAN_POINT('',(-36.5815530155254,28.5,-2199.54745691296));
#2417=CARTESIAN_POINT('Origin',(-36.5815530155254,30.,-1949.54745691296));
#2418=CARTESIAN_POINT('',(-36.5815530155254,28.5,-2179.54745691296));
#2419=CARTESIAN_POINT('',(-36.5815530155254,1.5,-2179.54745691296));
#2420=CARTESIAN_POINT('',(-36.5815530155254,30.,-2179.54745691296));
#2421=CARTESIAN_POINT('',(-36.5815530155254,1.5,-1969.54745691296));
#2422=CARTESIAN_POINT('',(-36.5815530155254,1.5,-1969.54745691296));
#2423=CARTESIAN_POINT('',(-36.5815530155254,28.5,-1969.54745691296));
#2424=CARTESIAN_POINT('',(-36.5815530155254,30.,-1969.54745691296));
#2425=CARTESIAN_POINT('',(-36.5815530155254,28.5,-1949.54745691296));
#2426=CARTESIAN_POINT('Origin',(-36.5815530155254,30.,-1949.54745691296));
#2427=CARTESIAN_POINT('',(-16.5815530155254,28.5,-1949.54745691296));
#2428=CARTESIAN_POINT('',(-16.5815530155254,1.5,-1949.54745691296));
#2429=CARTESIAN_POINT('',(-16.5815530155254,0.,-1949.54745691296));
#2430=CARTESIAN_POINT('',(193.418446984475,1.5,-1949.54745691296));
#2431=CARTESIAN_POINT('',(-36.5815530155254,1.5,-1949.54745691296));
#2432=CARTESIAN_POINT('',(193.418446984475,28.5,-1949.54745691296));
#2433=CARTESIAN_POINT('',(193.418446984475,30.,-1949.54745691296));
#2434=CARTESIAN_POINT('',(-16.5815530155254,28.5,-1949.54745691296));
#2435=CARTESIAN_POINT('Origin',(213.418446984475,30.,-1949.54745691296));
#2436=CARTESIAN_POINT('',(213.418446984475,1.5,-2179.54745691296));
#2437=CARTESIAN_POINT('',(213.418446984475,28.5,-2179.54745691296));
#2438=CARTESIAN_POINT('',(213.418446984475,30.,-2179.54745691296));
#2439=CARTESIAN_POINT('',(213.418446984475,28.5,-1969.54745691296));
#2440=CARTESIAN_POINT('',(213.418446984475,28.5,-1969.54745691296));
#2441=CARTESIAN_POINT('',(213.418446984475,1.5,-1969.54745691296));
#2442=CARTESIAN_POINT('',(213.418446984475,30.,-1969.54745691296));
#2443=CARTESIAN_POINT('',(213.418446984475,1.5,-1949.54745691296));
#2444=CARTESIAN_POINT('Origin',(0.,30.,0.));
#2445=CARTESIAN_POINT('',(-35.0815530155254,30.,-2179.54745691296));
#2446=CARTESIAN_POINT('',(-35.0815530155254,30.,-1969.54745691296));
#2447=CARTESIAN_POINT('',(-35.0815530155254,30.,0.));
#2448=CARTESIAN_POINT('',(-16.5815530155254,30.,-1951.04745691296));
#2449=CARTESIAN_POINT('Origin',(-16.5815530155254,30.,-1969.54745691296));
#2450=CARTESIAN_POINT('',(193.418446984475,30.,-1951.04745691296));
#2451=CARTESIAN_POINT('',(193.418446984475,30.,-1951.04745691296));
#2452=CARTESIAN_POINT('',(211.918446984475,30.,-1969.54745691296));
#2453=CARTESIAN_POINT('Origin',(193.418446984475,30.,-1969.54745691296));
#2454=CARTESIAN_POINT('',(211.918446984475,30.,-2179.54745691296));
#2455=CARTESIAN_POINT('',(211.918446984475,30.,-2179.54745691296));
#2456=CARTESIAN_POINT('',(193.418446984475,30.,-2198.04745691296));
#2457=CARTESIAN_POINT('Origin',(193.418446984475,30.,-2179.54745691296));
#2458=CARTESIAN_POINT('',(-16.5815530155254,30.,-2198.04745691296));
#2459=CARTESIAN_POINT('',(0.,30.,-2198.04745691296));
#2460=CARTESIAN_POINT('Origin',(-16.5815530155254,30.,-2179.54745691296));
#2461=CARTESIAN_POINT('Origin',(0.,0.,0.));
#2462=CARTESIAN_POINT('',(211.918446984475,0.,-2179.54745691296));
#2463=CARTESIAN_POINT('',(211.918446984475,0.,-1969.54745691296));
#2464=CARTESIAN_POINT('',(211.918446984475,0.,0.));
#2465=CARTESIAN_POINT('',(193.418446984475,0.,-1951.04745691296));
#2466=CARTESIAN_POINT('Origin',(193.418446984475,0.,-1969.54745691296));
#2467=CARTESIAN_POINT('',(-16.5815530155254,0.,-1951.04745691296));
#2468=CARTESIAN_POINT('',(0.,0.,-1951.04745691296));
#2469=CARTESIAN_POINT('',(-35.0815530155254,0.,-1969.54745691296));
#2470=CARTESIAN_POINT('Origin',(-16.5815530155254,0.,-1969.54745691296));
#2471=CARTESIAN_POINT('',(-35.0815530155254,0.,-2179.54745691296));
#2472=CARTESIAN_POINT('',(-35.0815530155254,0.,-2179.54745691296));
#2473=CARTESIAN_POINT('',(-16.5815530155254,0.,-2198.04745691296));
#2474=CARTESIAN_POINT('Origin',(-16.5815530155254,0.,-2179.54745691296));
#2475=CARTESIAN_POINT('',(193.418446984475,0.,-2198.04745691296));
#2476=CARTESIAN_POINT('',(193.418446984475,0.,-2198.04745691296));
#2477=CARTESIAN_POINT('Origin',(193.418446984475,0.,-2179.54745691296));
#2478=CARTESIAN_POINT('Origin',(-16.5815530155254,30.,-1969.54745691296));
#2479=CARTESIAN_POINT('Origin',(-16.5815530155254,1.5,-1969.54745691296));
#2480=CARTESIAN_POINT('Origin',(-16.5815530155254,28.5,-1969.54745691296));
#2481=CARTESIAN_POINT('Origin',(-16.5815530155254,30.,-2179.54745691296));
#2482=CARTESIAN_POINT('Origin',(-16.5815530155254,1.5,-2179.54745691296));
#2483=CARTESIAN_POINT('Origin',(-16.5815530155254,28.5,-2179.54745691296));
#2484=CARTESIAN_POINT('Origin',(193.418446984475,30.,-2179.54745691296));
#2485=CARTESIAN_POINT('Origin',(193.418446984475,1.5,-2179.54745691296));
#2486=CARTESIAN_POINT('Origin',(193.418446984475,28.5,-2179.54745691296));
#2487=CARTESIAN_POINT('Origin',(193.418446984475,30.,-1969.54745691296));
#2488=CARTESIAN_POINT('Origin',(193.418446984475,1.5,-1969.54745691296));
#2489=CARTESIAN_POINT('Origin',(193.418446984475,28.5,-1969.54745691296));
#2490=CARTESIAN_POINT('Origin',(-16.5815530155254,1.5,-2179.54745691296));
#2491=CARTESIAN_POINT('Origin',(-35.0815530155254,1.5,-2179.54745691296));
#2492=CARTESIAN_POINT('Origin',(-16.5815530155254,1.5,-2198.04745691296));
#2493=CARTESIAN_POINT('Origin',(0.,1.5,-2198.04745691296));
#2494=CARTESIAN_POINT('Origin',(193.418446984475,1.5,-2198.04745691296));
#2495=CARTESIAN_POINT('Origin',(-35.0815530155254,1.5,0.));
#2496=CARTESIAN_POINT('Origin',(-35.0815530155254,1.5,-1969.54745691296));
#2497=CARTESIAN_POINT('Origin',(193.418446984475,1.5,-2179.54745691296));
#2498=CARTESIAN_POINT('Origin',(211.918446984475,1.5,-2179.54745691296));
#2499=CARTESIAN_POINT('Origin',(-16.5815530155254,1.5,-1969.54745691296));
#2500=CARTESIAN_POINT('Origin',(-16.5815530155254,1.5,-1951.04745691296));
#2501=CARTESIAN_POINT('Origin',(211.918446984475,1.5,-1949.54745691296));
#2502=CARTESIAN_POINT('Origin',(211.918446984475,1.5,-1969.54745691296));
#2503=CARTESIAN_POINT('Origin',(-36.5815530155254,1.5,-1951.04745691296));
#2504=CARTESIAN_POINT('Origin',(193.418446984475,1.5,-1951.04745691296));
#2505=CARTESIAN_POINT('Origin',(193.418446984475,1.5,-1969.54745691296));
#2506=CARTESIAN_POINT('Origin',(193.418446984475,28.5,-2179.54745691296));
#2507=CARTESIAN_POINT('Origin',(211.918446984475,28.5,-2179.54745691296));
#2508=CARTESIAN_POINT('Origin',(193.418446984475,28.5,-2198.04745691296));
#2509=CARTESIAN_POINT('Origin',(-36.5815530155254,28.5,-2198.04745691296));
#2510=CARTESIAN_POINT('Origin',(-16.5815530155254,28.5,-2198.04745691296));
#2511=CARTESIAN_POINT('Origin',(211.918446984475,28.5,0.));
#2512=CARTESIAN_POINT('Origin',(211.918446984475,28.5,-1969.54745691296));
#2513=CARTESIAN_POINT('Origin',(-16.5815530155254,28.5,-2179.54745691296));
#2514=CARTESIAN_POINT('Origin',(-35.0815530155254,28.5,-2179.54745691296));
#2515=CARTESIAN_POINT('Origin',(193.418446984475,28.5,-1969.54745691296));
#2516=CARTESIAN_POINT('Origin',(193.418446984475,28.5,-1951.04745691296));
#2517=CARTESIAN_POINT('Origin',(-35.0815530155254,28.5,-1949.54745691296));
#2518=CARTESIAN_POINT('Origin',(-35.0815530155254,28.5,-1969.54745691296));
#2519=CARTESIAN_POINT('Origin',(0.,28.5,-1951.04745691296));
#2520=CARTESIAN_POINT('Origin',(-16.5815530155254,28.5,-1951.04745691296));
#2521=CARTESIAN_POINT('Origin',(-16.5815530155254,28.5,-1969.54745691296));
#2522=CARTESIAN_POINT('Origin',(88.4184469844746,20.,-2074.54745691296));
#2826=UNCERTAINTY_MEASURE_WITH_UNIT(LENGTH_MEASURE(0.01),#2841,
'DISTANCE_ACCURACY_VALUE',
'Maximum model space distance between geometric entities at asserted c
onnectivities');
#2832=UNCERTAINTY_MEASURE_WITH_UNIT(LENGTH_MEASURE(0.01),#2841,
'DISTANCE_ACCURACY_VALUE',
'Maximum model space distance between geometric entities at asserted c
onnectivities');
#2834=(
GEOMETRIC_REPRESENTATION_CONTEXT(3)
GLOBAL_UNCERTAINTY_ASSIGNED_CONTEXT((#2826))
GLOBAL_UNIT_ASSIGNED_CONTEXT((#2841,#2843,#2844))
REPRESENTATION_CONTEXT('','3D')
);
#2840=(
GEOMETRIC_REPRESENTATION_CONTEXT(3)
GLOBAL_UNCERTAINTY_ASSIGNED_CONTEXT((#2832))
GLOBAL_UNIT_ASSIGNED_CONTEXT((#2841,#2843,#2844))
REPRESENTATION_CONTEXT('','3D')
);
#2841=(
LENGTH_UNIT()
NAMED_UNIT(*)
SI_UNIT(.MILLI.,.METRE.)
);
#2843=(
NAMED_UNIT(*)
PLANE_ANGLE_UNIT()
SI_UNIT($,.RADIAN.)
);
#2844=(
NAMED_UNIT(*)
SI_UNIT($,.STERADIAN.)
SOLID_ANGLE_UNIT()
);
#2846=SHAPE_DEFINITION_REPRESENTATION(#2853,#2866);
#2853=PRODUCT_DEFINITION_SHAPE('',$,#2874);
#2866=SHAPE_REPRESENTATION('',(#1621),#2834);
#2872=PRODUCT_DEFINITION_CONTEXT('part definition',#2895,'design');
#2874=PRODUCT_DEFINITION('BASE PLATE','BASE PLATE',#2881,#2872);
#2881=PRODUCT_DEFINITION_FORMATION('',$,#2898);
#2895=APPLICATION_CONTEXT(
'Core Data for Automotive Mechanical Design Process');
#2896=PRODUCT_CONTEXT('part definition',#2895,'mechanical');
#2898=PRODUCT('BASE PLATE','BASE PLATE',$,(#2896));
#2905=PRESENTATION_STYLE_ASSIGNMENT((#2907));
#2907=SURFACE_STYLE_USAGE(.BOTH.,#2909);
#2909=SURFACE_SIDE_STYLE('',(#2911));
#2911=SURFACE_STYLE_FILL_AREA(#2913);
#2913=FILL_AREA_STYLE('Opaque(202,209,238)',(#2915));
#2915=FILL_AREA_STYLE_COLOUR('Opaque(202,209,238)',#2917);
#2917=COLOUR_RGB('Opaque(202,209,238)', 0.66274510, 0.83137255, 0.94901961);
ENDSEC;
END-ISO-10303-21;
